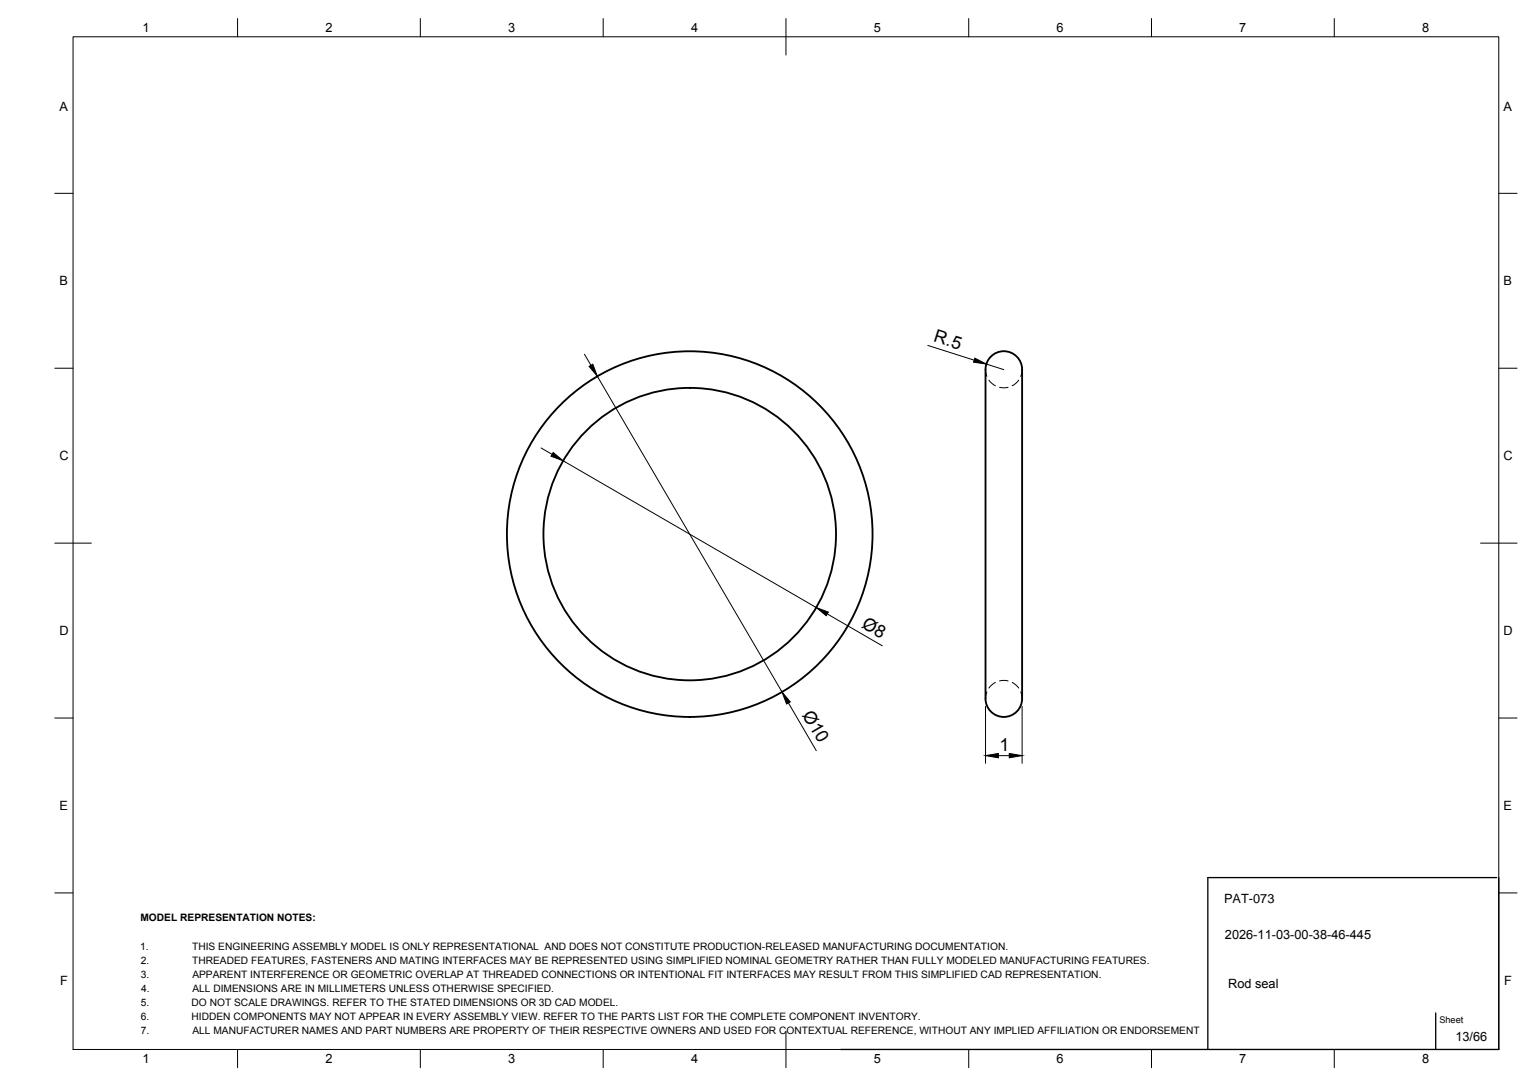
ISO-10303-21;
HEADER;
/* Generated by software containing ST-Developer
 * from STEP Tools, Inc. (www.steptools.com) 
 */

FILE_DESCRIPTION(
/* description */ ('Manual piston pump'),
/* implementation_level */ '2;1');

FILE_NAME(
/* name */ 'Rod seal.step',
/* time_stamp */ '2026-11-02T16:54:23-08:00',
/* author */ (''),
/* organization */ (''),
/* preprocessor_version */ 'ST-DEVELOPER v20.2',
/* originating_system */ 'Autodesk Translation Framework v15.17.0.0',
/* authorisation */ '');

FILE_SCHEMA (('AUTOMOTIVE_DESIGN { 1 0 10303 214 3 1 1 }'));
ENDSEC;

DATA;
#10=MECHANICAL_DESIGN_GEOMETRIC_PRESENTATION_REPRESENTATION('',(#696),#19043);
#558=TOROIDAL_SURFACE('',#10450,0.45,0.05);
#570=SHAPE_REPRESENTATION_RELATIONSHIP('SRR','None',#19316,#633);
#633=ADVANCED_BREP_SHAPE_REPRESENTATION('',(#768),#18983);
#696=STYLED_ITEM('',(#19661),#768);
#768=MANIFOLD_SOLID_BREP('Body1',#9480);
#1392=FACE_OUTER_BOUND('',#2024,.T.);
#2024=EDGE_LOOP('',(#6707,#6708,#6709,#6710));
#2759=CIRCLE('',#10451,0.05);
#2760=CIRCLE('',#10452,0.4);
#4499=VERTEX_POINT('',#15127);
#5340=EDGE_CURVE('',#4499,#4499,#2759,.T.);
#5341=EDGE_CURVE('',#4499,#4499,#2760,.T.);
#6707=ORIENTED_EDGE('',*,*,#5340,.F.);
#6708=ORIENTED_EDGE('',*,*,#5341,.T.);
#6709=ORIENTED_EDGE('',*,*,#5340,.T.);
#6710=ORIENTED_EDGE('',*,*,#5341,.F.);
#8997=ADVANCED_FACE('',(#1392),#558,.T.);
#9480=CLOSED_SHELL('',(#8997));
#10449=AXIS2_PLACEMENT_3D('',#15125,#12025,#12026);
#10450=AXIS2_PLACEMENT_3D('',#15126,#12027,#12028);
#10451=AXIS2_PLACEMENT_3D('',#15128,#12029,#12030);
#10452=AXIS2_PLACEMENT_3D('',#15129,#12031,#12032);
#12025=DIRECTION('axis',(0.,0.,1.));
#12026=DIRECTION('refdir',(1.,0.,0.));
#12027=DIRECTION('center_axis',(0.,-1.,0.));
#12028=DIRECTION('ref_axis',(0.,0.,-1.));
#12029=DIRECTION('center_axis',(-1.,0.,-1.22464679914735E-16));
#12030=DIRECTION('ref_axis',(-1.22464679914735E-16,0.,1.));
#12031=DIRECTION('center_axis',(0.,1.,0.));
#12032=DIRECTION('ref_axis',(0.,0.,-1.));
#15125=CARTESIAN_POINT('',(0.,0.,0.));
#15126=CARTESIAN_POINT('Origin',(0.,0.2,4.5));
#15127=CARTESIAN_POINT('',(-4.89858719658941E-17,0.2,4.9));
#15128=CARTESIAN_POINT('Origin',(-5.51091059616309E-17,0.2,4.95));
#15129=CARTESIAN_POINT('Origin',(0.,0.2,4.5));
#18912=UNCERTAINTY_MEASURE_WITH_UNIT(LENGTH_MEASURE(0.001),#19044,
'DISTANCE_ACCURACY_VALUE',
'Maximum model space distance between geometric entities at asserted c
onnectivities');
#18972=UNCERTAINTY_MEASURE_WITH_UNIT(LENGTH_MEASURE(0.001),#19044,
'DISTANCE_ACCURACY_VALUE',
'Maximum model space distance between geometric entities at asserted c
onnectivities');
#18983=(
GEOMETRIC_REPRESENTATION_CONTEXT(3)
GLOBAL_UNCERTAINTY_ASSIGNED_CONTEXT((#18912))
GLOBAL_UNIT_ASSIGNED_CONTEXT((#19044,#19046,#19047))
REPRESENTATION_CONTEXT('','3D')
);
#19043=(
GEOMETRIC_REPRESENTATION_CONTEXT(3)
GLOBAL_UNCERTAINTY_ASSIGNED_CONTEXT((#18972))
GLOBAL_UNIT_ASSIGNED_CONTEXT((#19044,#19046,#19047))
REPRESENTATION_CONTEXT('','3D')
);
#19044=(
LENGTH_UNIT()
NAMED_UNIT(*)
SI_UNIT(.CENTI.,.METRE.)
);
#19046=(
NAMED_UNIT(*)
PLANE_ANGLE_UNIT()
SI_UNIT($,.RADIAN.)
);
#19047=(
NAMED_UNIT(*)
SI_UNIT($,.STERADIAN.)
SOLID_ANGLE_UNIT()
);
#19058=SHAPE_DEFINITION_REPRESENTATION(#19128,#19316);
#19128=PRODUCT_DEFINITION_SHAPE('',$,#19387);
#19316=SHAPE_REPRESENTATION('',(#10449),#18983);
#19376=PRODUCT_DEFINITION_CONTEXT('part definition',#19588,'design');
#19387=PRODUCT_DEFINITION('2026-11-03-00-38-46-445','Rod seal',#19457,#19376);
#19457=PRODUCT_DEFINITION_FORMATION('',$,#19600);
#19588=APPLICATION_CONTEXT(
'Core Data for Automotive Mechanical Design Process');
#19589=PRODUCT_CONTEXT('part definition',#19588,'mechanical');
#19600=PRODUCT('2026-11-03-00-38-46-445','Rod seal','Rod seal',(#19589));
#19661=PRESENTATION_STYLE_ASSIGNMENT((#19667));
#19667=SURFACE_STYLE_USAGE(.BOTH.,#19673);
#19673=SURFACE_SIDE_STYLE('',(#19679));
#19679=SURFACE_STYLE_FILL_AREA(#19685);
#19685=FILL_AREA_STYLE('CAD Library Painted - Engineering blue',(#19691));
#19691=FILL_AREA_STYLE_COLOUR('CAD Library Painted - Engineering blue',
#19697);
#19697=COLOUR_RGB('CAD Library Painted - Engineering blue',0.12156862745098,
0.356862745098039,0.6);
ENDSEC;
END-ISO-10303-21;
